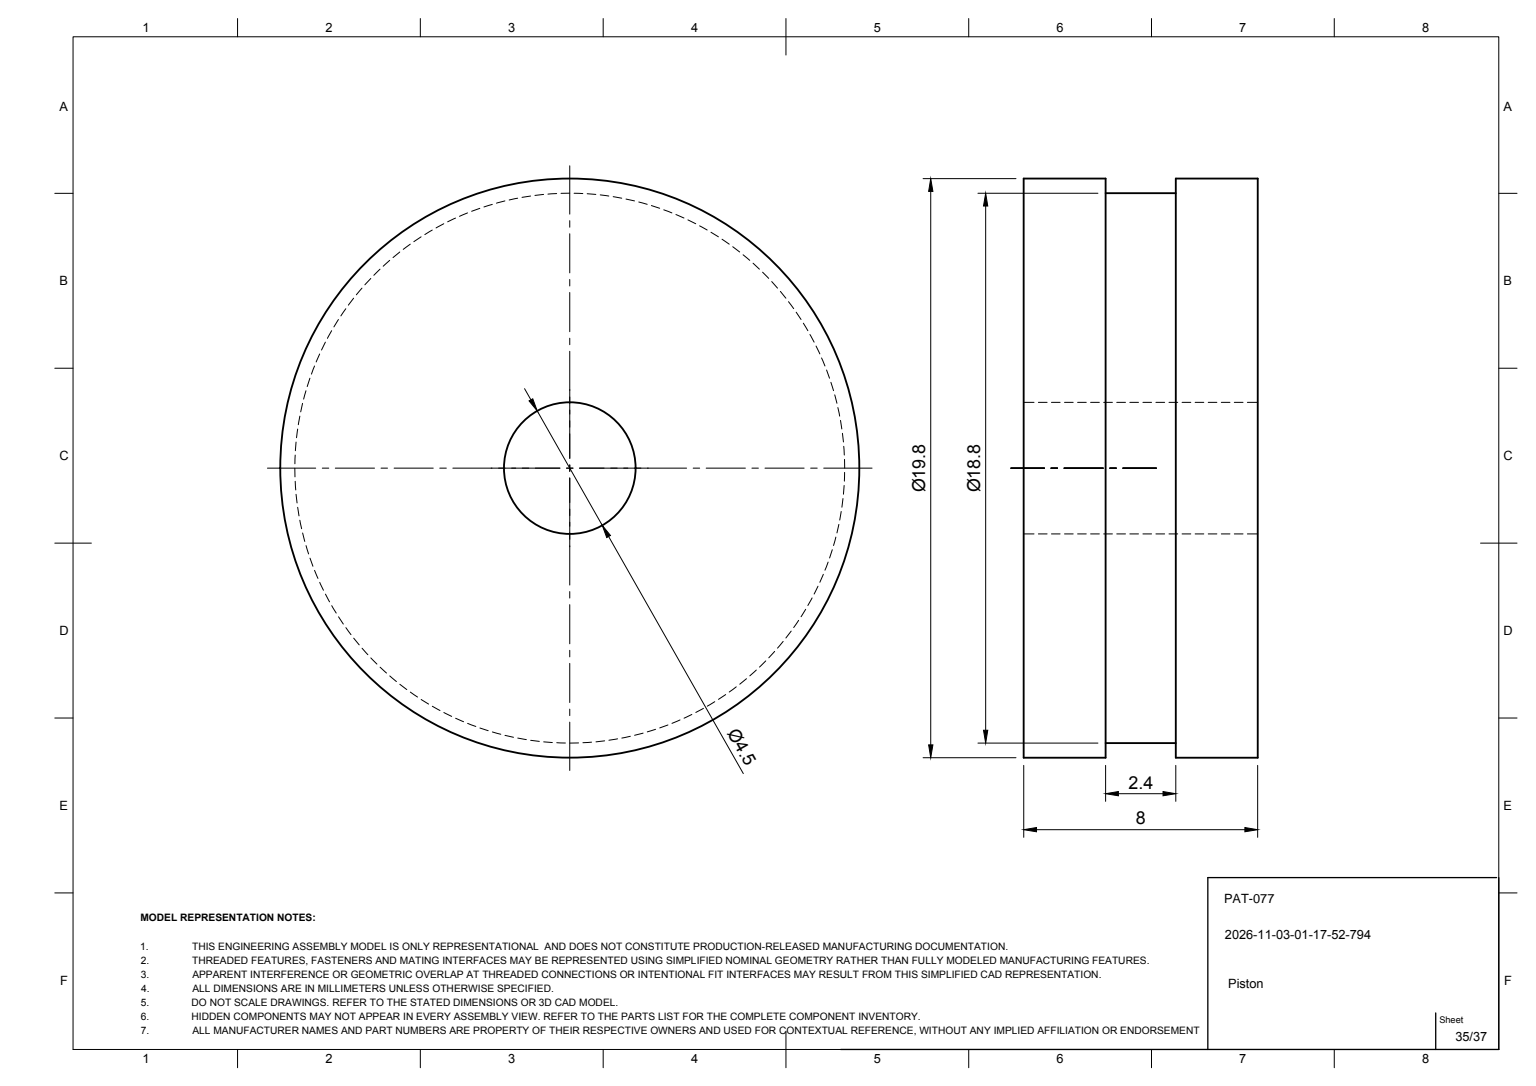
ISO-10303-21;
HEADER;
/* Generated by software containing ST-Developer
 * from STEP Tools, Inc. (www.steptools.com) 
 */

FILE_DESCRIPTION(
/* description */ ('Pallet stop with pneumatic fitting'),
/* implementation_level */ '2;1');

FILE_NAME(
/* name */ 'Piston.step',
/* time_stamp */ '2026-10-27T10:51:41-07:00',
/* author */ (''),
/* organization */ (''),
/* preprocessor_version */ 'ST-DEVELOPER v20.2',
/* originating_system */ 'Autodesk Translation Framework v15.17.0.0',
/* authorisation */ '');

FILE_SCHEMA (('AUTOMOTIVE_DESIGN { 1 0 10303 214 3 1 1 }'));
ENDSEC;

DATA;
#10=MECHANICAL_DESIGN_GEOMETRIC_PRESENTATION_REPRESENTATION('',(#384),#10265);
#320=SHAPE_REPRESENTATION_RELATIONSHIP('SRR','None',#10436,#352);
#352=ADVANCED_BREP_SHAPE_REPRESENTATION('',(#415),#10260);
#384=STYLED_ITEM('',(#10648),#415);
#415=MANIFOLD_SOLID_BREP('Body1',#5073);
#537=FACE_BOUND('',#1440,.T.);
#538=FACE_BOUND('',#1442,.T.);
#539=FACE_BOUND('',#1447,.T.);
#540=FACE_BOUND('',#1449,.T.);
#708=PLANE('',#5962);
#709=PLANE('',#5964);
#710=PLANE('',#5973);
#711=PLANE('',#5974);
#1006=FACE_OUTER_BOUND('',#1438,.T.);
#1007=FACE_OUTER_BOUND('',#1439,.T.);
#1008=FACE_OUTER_BOUND('',#1441,.T.);
#1009=FACE_OUTER_BOUND('',#1443,.T.);
#1010=FACE_OUTER_BOUND('',#1444,.T.);
#1011=FACE_OUTER_BOUND('',#1445,.T.);
#1012=FACE_OUTER_BOUND('',#1446,.T.);
#1013=FACE_OUTER_BOUND('',#1448,.T.);
#1438=EDGE_LOOP('',(#4466,#4467,#4468,#4469));
#1439=EDGE_LOOP('',(#4470));
#1440=EDGE_LOOP('',(#4471));
#1441=EDGE_LOOP('',(#4472));
#1442=EDGE_LOOP('',(#4473));
#1443=EDGE_LOOP('',(#4474,#4475,#4476,#4477));
#1444=EDGE_LOOP('',(#4478,#4479,#4480,#4481));
#1445=EDGE_LOOP('',(#4482,#4483,#4484,#4485));
#1446=EDGE_LOOP('',(#4486));
#1447=EDGE_LOOP('',(#4487));
#1448=EDGE_LOOP('',(#4488));
#1449=EDGE_LOOP('',(#4489));
#1773=LINE('',#9962,#2108);
#1774=LINE('',#9972,#2109);
#1775=LINE('',#9978,#2110);
#1776=LINE('',#9983,#2111);
#2108=VECTOR('',#7430,0.94);
#2109=VECTOR('',#7443,0.99);
#2110=VECTOR('',#7450,0.225);
#2111=VECTOR('',#7457,0.99);
#2381=CIRCLE('',#5960,0.94);
#2382=CIRCLE('',#5961,0.94);
#2383=CIRCLE('',#5963,0.99);
#2384=CIRCLE('',#5965,0.99);
#2385=CIRCLE('',#5967,0.99);
#2386=CIRCLE('',#5969,0.225);
#2387=CIRCLE('',#5970,0.225);
#2388=CIRCLE('',#5972,0.99);
#2754=VERTEX_POINT('',#9959);
#2755=VERTEX_POINT('',#9961);
#2756=VERTEX_POINT('',#9965);
#2757=VERTEX_POINT('',#9968);
#2758=VERTEX_POINT('',#9971);
#2759=VERTEX_POINT('',#9975);
#2760=VERTEX_POINT('',#9977);
#2761=VERTEX_POINT('',#9981);
#3332=EDGE_CURVE('',#2754,#2754,#2381,.T.);
#3333=EDGE_CURVE('',#2754,#2755,#1773,.T.);
#3334=EDGE_CURVE('',#2755,#2755,#2382,.T.);
#3335=EDGE_CURVE('',#2756,#2756,#2383,.T.);
#3336=EDGE_CURVE('',#2757,#2757,#2384,.T.);
#3337=EDGE_CURVE('',#2757,#2758,#1774,.T.);
#3338=EDGE_CURVE('',#2758,#2758,#2385,.T.);
#3339=EDGE_CURVE('',#2759,#2759,#2386,.T.);
#3340=EDGE_CURVE('',#2759,#2760,#1775,.T.);
#3341=EDGE_CURVE('',#2760,#2760,#2387,.T.);
#3342=EDGE_CURVE('',#2761,#2761,#2388,.T.);
#3343=EDGE_CURVE('',#2761,#2756,#1776,.T.);
#4466=ORIENTED_EDGE('',*,*,#3332,.F.);
#4467=ORIENTED_EDGE('',*,*,#3333,.T.);
#4468=ORIENTED_EDGE('',*,*,#3334,.T.);
#4469=ORIENTED_EDGE('',*,*,#3333,.F.);
#4470=ORIENTED_EDGE('',*,*,#3335,.F.);
#4471=ORIENTED_EDGE('',*,*,#3334,.F.);
#4472=ORIENTED_EDGE('',*,*,#3336,.F.);
#4473=ORIENTED_EDGE('',*,*,#3332,.T.);
#4474=ORIENTED_EDGE('',*,*,#3336,.T.);
#4475=ORIENTED_EDGE('',*,*,#3337,.T.);
#4476=ORIENTED_EDGE('',*,*,#3338,.T.);
#4477=ORIENTED_EDGE('',*,*,#3337,.F.);
#4478=ORIENTED_EDGE('',*,*,#3339,.F.);
#4479=ORIENTED_EDGE('',*,*,#3340,.T.);
#4480=ORIENTED_EDGE('',*,*,#3341,.T.);
#4481=ORIENTED_EDGE('',*,*,#3340,.F.);
#4482=ORIENTED_EDGE('',*,*,#3342,.F.);
#4483=ORIENTED_EDGE('',*,*,#3343,.T.);
#4484=ORIENTED_EDGE('',*,*,#3335,.T.);
#4485=ORIENTED_EDGE('',*,*,#3343,.F.);
#4486=ORIENTED_EDGE('',*,*,#3342,.T.);
#4487=ORIENTED_EDGE('',*,*,#3339,.T.);
#4488=ORIENTED_EDGE('',*,*,#3338,.F.);
#4489=ORIENTED_EDGE('',*,*,#3341,.F.);
#4721=CYLINDRICAL_SURFACE('',#5959,0.94);
#4722=CYLINDRICAL_SURFACE('',#5966,0.99);
#4723=CYLINDRICAL_SURFACE('',#5968,0.225);
#4724=CYLINDRICAL_SURFACE('',#5971,0.99);
#5001=ADVANCED_FACE('',(#1006),#4721,.T.);
#5002=ADVANCED_FACE('',(#1007,#537),#708,.F.);
#5003=ADVANCED_FACE('',(#1008,#538),#709,.T.);
#5004=ADVANCED_FACE('',(#1009),#4722,.T.);
#5005=ADVANCED_FACE('',(#1010),#4723,.F.);
#5006=ADVANCED_FACE('',(#1011),#4724,.T.);
#5007=ADVANCED_FACE('',(#1012,#539),#710,.T.);
#5008=ADVANCED_FACE('',(#1013,#540),#711,.F.);
#5073=CLOSED_SHELL('',(#5001,#5002,#5003,#5004,#5005,#5006,#5007,#5008));
#5958=AXIS2_PLACEMENT_3D('',#9957,#7424,#7425);
#5959=AXIS2_PLACEMENT_3D('',#9958,#7426,#7427);
#5960=AXIS2_PLACEMENT_3D('',#9960,#7428,#7429);
#5961=AXIS2_PLACEMENT_3D('',#9963,#7431,#7432);
#5962=AXIS2_PLACEMENT_3D('',#9964,#7433,#7434);
#5963=AXIS2_PLACEMENT_3D('',#9966,#7435,#7436);
#5964=AXIS2_PLACEMENT_3D('',#9967,#7437,#7438);
#5965=AXIS2_PLACEMENT_3D('',#9969,#7439,#7440);
#5966=AXIS2_PLACEMENT_3D('',#9970,#7441,#7442);
#5967=AXIS2_PLACEMENT_3D('',#9973,#7444,#7445);
#5968=AXIS2_PLACEMENT_3D('',#9974,#7446,#7447);
#5969=AXIS2_PLACEMENT_3D('',#9976,#7448,#7449);
#5970=AXIS2_PLACEMENT_3D('',#9979,#7451,#7452);
#5971=AXIS2_PLACEMENT_3D('',#9980,#7453,#7454);
#5972=AXIS2_PLACEMENT_3D('',#9982,#7455,#7456);
#5973=AXIS2_PLACEMENT_3D('',#9984,#7458,#7459);
#5974=AXIS2_PLACEMENT_3D('',#9985,#7460,#7461);
#7424=DIRECTION('axis',(0.,0.,1.));
#7425=DIRECTION('refdir',(1.,0.,0.));
#7426=DIRECTION('center_axis',(0.,0.,1.));
#7427=DIRECTION('ref_axis',(1.,0.,0.));
#7428=DIRECTION('center_axis',(0.,0.,-1.));
#7429=DIRECTION('ref_axis',(1.,0.,0.));
#7430=DIRECTION('',(0.,0.,1.));
#7431=DIRECTION('center_axis',(0.,0.,-1.));
#7432=DIRECTION('ref_axis',(1.,0.,0.));
#7433=DIRECTION('center_axis',(0.,0.,1.));
#7434=DIRECTION('ref_axis',(1.,0.,0.));
#7435=DIRECTION('center_axis',(0.,0.,1.));
#7436=DIRECTION('ref_axis',(1.,0.,0.));
#7437=DIRECTION('center_axis',(0.,0.,1.));
#7438=DIRECTION('ref_axis',(1.,0.,0.));
#7439=DIRECTION('center_axis',(0.,0.,-1.));
#7440=DIRECTION('ref_axis',(1.,0.,0.));
#7441=DIRECTION('center_axis',(0.,0.,1.));
#7442=DIRECTION('ref_axis',(1.,0.,0.));
#7443=DIRECTION('',(0.,0.,-1.));
#7444=DIRECTION('center_axis',(0.,0.,1.));
#7445=DIRECTION('ref_axis',(1.,0.,0.));
#7446=DIRECTION('center_axis',(0.,0.,1.));
#7447=DIRECTION('ref_axis',(1.,0.,0.));
#7448=DIRECTION('center_axis',(0.,0.,-1.));
#7449=DIRECTION('ref_axis',(1.,0.,0.));
#7450=DIRECTION('',(0.,0.,-1.));
#7451=DIRECTION('center_axis',(0.,0.,-1.));
#7452=DIRECTION('ref_axis',(1.,0.,0.));
#7453=DIRECTION('center_axis',(0.,0.,1.));
#7454=DIRECTION('ref_axis',(1.,0.,0.));
#7455=DIRECTION('center_axis',(0.,0.,1.));
#7456=DIRECTION('ref_axis',(1.,0.,0.));
#7457=DIRECTION('',(0.,0.,-1.));
#7458=DIRECTION('center_axis',(0.,0.,1.));
#7459=DIRECTION('ref_axis',(1.,0.,0.));
#7460=DIRECTION('center_axis',(0.,0.,1.));
#7461=DIRECTION('ref_axis',(1.,0.,0.));
#9957=CARTESIAN_POINT('',(0.,0.,0.));
#9958=CARTESIAN_POINT('Origin',(4.,4.,7.28));
#9959=CARTESIAN_POINT('',(3.06,4.,7.28));
#9960=CARTESIAN_POINT('Origin',(4.,4.,7.28));
#9961=CARTESIAN_POINT('',(3.06,4.,7.52));
#9962=CARTESIAN_POINT('',(3.06,4.,7.28));
#9963=CARTESIAN_POINT('Origin',(4.,4.,7.52));
#9964=CARTESIAN_POINT('Origin',(4.,4.,7.52));
#9965=CARTESIAN_POINT('',(3.01,4.,7.52));
#9966=CARTESIAN_POINT('Origin',(4.,4.,7.52));
#9967=CARTESIAN_POINT('Origin',(4.,4.,7.28));
#9968=CARTESIAN_POINT('',(3.01,4.,7.28));
#9969=CARTESIAN_POINT('Origin',(4.,4.,7.28));
#9970=CARTESIAN_POINT('Origin',(4.,4.,7.));
#9971=CARTESIAN_POINT('',(3.01,4.,7.));
#9972=CARTESIAN_POINT('',(3.01,4.,7.));
#9973=CARTESIAN_POINT('Origin',(4.,4.,7.));
#9974=CARTESIAN_POINT('Origin',(4.,4.,7.));
#9975=CARTESIAN_POINT('',(3.775,4.,7.8));
#9976=CARTESIAN_POINT('Origin',(4.,4.,7.8));
#9977=CARTESIAN_POINT('',(3.775,4.,7.));
#9978=CARTESIAN_POINT('',(3.775,4.,7.));
#9979=CARTESIAN_POINT('Origin',(4.,4.,7.));
#9980=CARTESIAN_POINT('Origin',(4.,4.,7.));
#9981=CARTESIAN_POINT('',(3.01,4.,7.8));
#9982=CARTESIAN_POINT('Origin',(4.,4.,7.8));
#9983=CARTESIAN_POINT('',(3.01,4.,7.));
#9984=CARTESIAN_POINT('Origin',(4.,4.,7.8));
#9985=CARTESIAN_POINT('Origin',(4.,4.,7.));
#10222=UNCERTAINTY_MEASURE_WITH_UNIT(LENGTH_MEASURE(0.001),#10266,
'DISTANCE_ACCURACY_VALUE',
'Maximum model space distance between geometric entities at asserted c
onnectivities');
#10227=UNCERTAINTY_MEASURE_WITH_UNIT(LENGTH_MEASURE(0.001),#10266,
'DISTANCE_ACCURACY_VALUE',
'Maximum model space distance between geometric entities at asserted c
onnectivities');
#10260=(
GEOMETRIC_REPRESENTATION_CONTEXT(3)
GLOBAL_UNCERTAINTY_ASSIGNED_CONTEXT((#10222))
GLOBAL_UNIT_ASSIGNED_CONTEXT((#10266,#10268,#10269))
REPRESENTATION_CONTEXT('','3D')
);
#10265=(
GEOMETRIC_REPRESENTATION_CONTEXT(3)
GLOBAL_UNCERTAINTY_ASSIGNED_CONTEXT((#10227))
GLOBAL_UNIT_ASSIGNED_CONTEXT((#10266,#10268,#10269))
REPRESENTATION_CONTEXT('','3D')
);
#10266=(
LENGTH_UNIT()
NAMED_UNIT(*)
SI_UNIT(.CENTI.,.METRE.)
);
#10268=(
NAMED_UNIT(*)
PLANE_ANGLE_UNIT()
SI_UNIT($,.RADIAN.)
);
#10269=(
NAMED_UNIT(*)
SI_UNIT($,.STERADIAN.)
SOLID_ANGLE_UNIT()
);
#10302=SHAPE_DEFINITION_REPRESENTATION(#10343,#10436);
#10343=PRODUCT_DEFINITION_SHAPE('',$,#10474);
#10436=SHAPE_REPRESENTATION('',(#5958),#10260);
#10441=PRODUCT_DEFINITION_CONTEXT('part definition',#10554,'design');
#10474=PRODUCT_DEFINITION('Piston','Piston',#10511,#10441);
#10511=PRODUCT_DEFINITION_FORMATION('',$,#10588);
#10554=APPLICATION_CONTEXT(
'Core Data for Automotive Mechanical Design Process');
#10555=PRODUCT_CONTEXT('part definition',#10554,'mechanical');
#10588=PRODUCT('Piston','Piston','Piston',(#10555));
#10642=COLOUR_RGB('Sky Blue',0.24,0.69,0.87);
#10643=FILL_AREA_STYLE_COLOUR('',#10642);
#10644=FILL_AREA_STYLE('',(#10643));
#10645=SURFACE_STYLE_FILL_AREA(#10644);
#10646=SURFACE_SIDE_STYLE('',(#10645));
#10647=SURFACE_STYLE_USAGE(.BOTH.,#10646);
#10648=PRESENTATION_STYLE_ASSIGNMENT((#10647));
ENDSEC;
END-ISO-10303-21;
